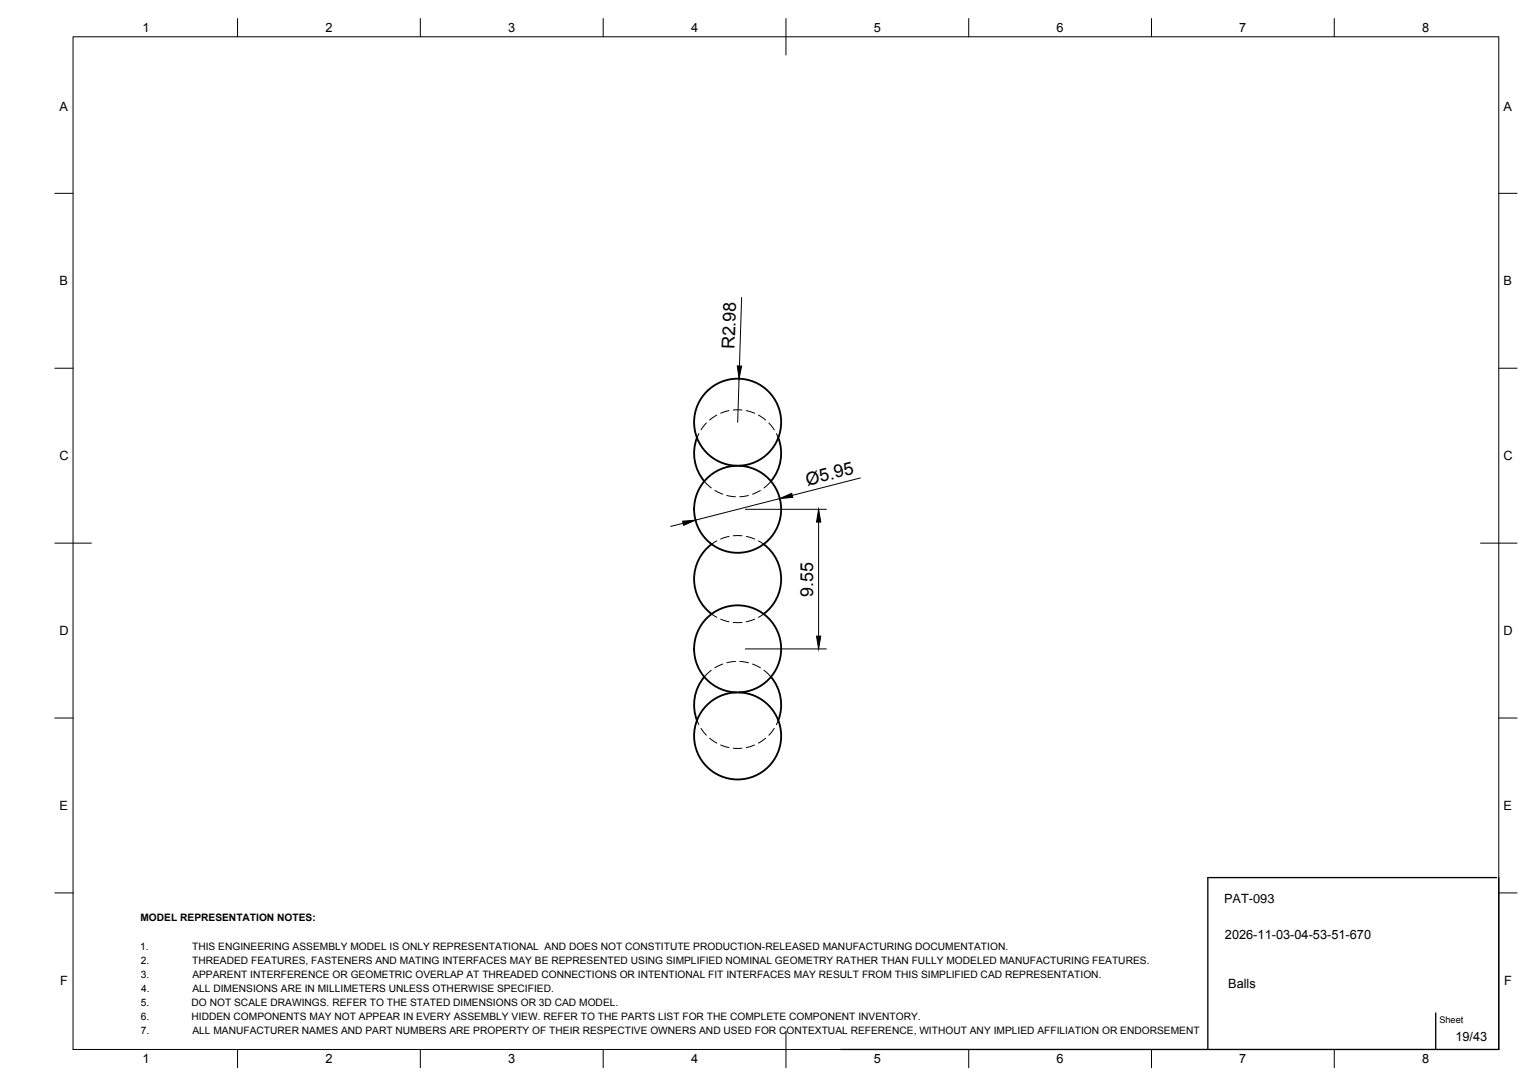
ISO-10303-21;
HEADER;
/* Generated by software containing ST-Developer
 * from STEP Tools, Inc. (www.steptools.com) 
 */

FILE_DESCRIPTION(
/* description */ ('Self-centering screw clamp'),
/* implementation_level */ '2;1');

FILE_NAME(
/* name */ 'Balls.step',
/* time_stamp */ '2026-10-28T03:25:31-07:00',
/* author */ (''),
/* organization */ (''),
/* preprocessor_version */ 'ST-DEVELOPER v20.2',
/* originating_system */ 'Autodesk Translation Framework v15.17.0.0',
/* authorisation */ '');

FILE_SCHEMA (('AUTOMOTIVE_DESIGN { 1 0 10303 214 3 1 1 }'));
ENDSEC;

DATA;
#10=MECHANICAL_DESIGN_GEOMETRIC_PRESENTATION_REPRESENTATION('',(#640,#641,#642,#643,#644,#645,#646),#16799);
#467=SPHERICAL_SURFACE('',#9996,0.29765);
#468=SPHERICAL_SURFACE('',#9998,0.29765);
#469=SPHERICAL_SURFACE('',#10000,0.29765);
#470=SPHERICAL_SURFACE('',#10002,0.29765);
#471=SPHERICAL_SURFACE('',#10004,0.29765);
#472=SPHERICAL_SURFACE('',#10006,0.29765);
#473=SPHERICAL_SURFACE('',#10008,0.29765);
#558=SHAPE_REPRESENTATION_RELATIONSHIP('SRR','None',#17032,#599);
#599=ADVANCED_BREP_SHAPE_REPRESENTATION('',(#688,#689,#690,#691,#692,#693,
#694),#16770);
#640=STYLED_ITEM('',(#17326),#688);
#641=STYLED_ITEM('',(#17326),#689);
#642=STYLED_ITEM('',(#17326),#690);
#643=STYLED_ITEM('',(#17326),#691);
#644=STYLED_ITEM('',(#17326),#692);
#645=STYLED_ITEM('',(#17326),#693);
#646=STYLED_ITEM('',(#17326),#694);
#688=MANIFOLD_SOLID_BREP('Body1',#9091);
#689=MANIFOLD_SOLID_BREP('Body2',#9092);
#690=MANIFOLD_SOLID_BREP('Body3',#9093);
#691=MANIFOLD_SOLID_BREP('Body4',#9094);
#692=MANIFOLD_SOLID_BREP('Body5',#9095);
#693=MANIFOLD_SOLID_BREP('Body6',#9096);
#694=MANIFOLD_SOLID_BREP('Body7',#9097);
#1470=FACE_OUTER_BOUND('',#2102,.T.);
#1471=FACE_OUTER_BOUND('',#2103,.T.);
#1472=FACE_OUTER_BOUND('',#2104,.T.);
#1473=FACE_OUTER_BOUND('',#2105,.T.);
#1474=FACE_OUTER_BOUND('',#2106,.T.);
#1475=FACE_OUTER_BOUND('',#2107,.T.);
#1476=FACE_OUTER_BOUND('',#2108,.T.);
#2102=EDGE_LOOP('',(#7057,#7058));
#2103=EDGE_LOOP('',(#7059,#7060));
#2104=EDGE_LOOP('',(#7061,#7062));
#2105=EDGE_LOOP('',(#7063,#7064));
#2106=EDGE_LOOP('',(#7065,#7066));
#2107=EDGE_LOOP('',(#7067,#7068));
#2108=EDGE_LOOP('',(#7069,#7070));
#3925=CIRCLE('',#9997,0.29765);
#3926=CIRCLE('',#9999,0.29765);
#3927=CIRCLE('',#10001,0.29765);
#3928=CIRCLE('',#10003,0.29765);
#3929=CIRCLE('',#10005,0.29765);
#3930=CIRCLE('',#10007,0.29765);
#3931=CIRCLE('',#10009,0.29765);
#4537=VERTEX_POINT('',#14754);
#4538=VERTEX_POINT('',#14755);
#4539=VERTEX_POINT('',#14758);
#4540=VERTEX_POINT('',#14759);
#4541=VERTEX_POINT('',#14762);
#4542=VERTEX_POINT('',#14763);
#4543=VERTEX_POINT('',#14766);
#4544=VERTEX_POINT('',#14767);
#4545=VERTEX_POINT('',#14770);
#4546=VERTEX_POINT('',#14771);
#4547=VERTEX_POINT('',#14774);
#4548=VERTEX_POINT('',#14775);
#4549=VERTEX_POINT('',#14778);
#4550=VERTEX_POINT('',#14779);
#5453=EDGE_CURVE('',#4537,#4538,#3925,.T.);
#5454=EDGE_CURVE('',#4539,#4540,#3926,.T.);
#5455=EDGE_CURVE('',#4541,#4542,#3927,.T.);
#5456=EDGE_CURVE('',#4543,#4544,#3928,.T.);
#5457=EDGE_CURVE('',#4545,#4546,#3929,.T.);
#5458=EDGE_CURVE('',#4547,#4548,#3930,.T.);
#5459=EDGE_CURVE('',#4549,#4550,#3931,.T.);
#7057=ORIENTED_EDGE('',*,*,#5453,.T.);
#7058=ORIENTED_EDGE('',*,*,#5453,.F.);
#7059=ORIENTED_EDGE('',*,*,#5454,.T.);
#7060=ORIENTED_EDGE('',*,*,#5454,.F.);
#7061=ORIENTED_EDGE('',*,*,#5455,.T.);
#7062=ORIENTED_EDGE('',*,*,#5455,.F.);
#7063=ORIENTED_EDGE('',*,*,#5456,.T.);
#7064=ORIENTED_EDGE('',*,*,#5456,.F.);
#7065=ORIENTED_EDGE('',*,*,#5457,.T.);
#7066=ORIENTED_EDGE('',*,*,#5457,.F.);
#7067=ORIENTED_EDGE('',*,*,#5458,.T.);
#7068=ORIENTED_EDGE('',*,*,#5458,.F.);
#7069=ORIENTED_EDGE('',*,*,#5459,.T.);
#7070=ORIENTED_EDGE('',*,*,#5459,.F.);
#8768=ADVANCED_FACE('',(#1470),#467,.T.);
#8769=ADVANCED_FACE('',(#1471),#468,.T.);
#8770=ADVANCED_FACE('',(#1472),#469,.T.);
#8771=ADVANCED_FACE('',(#1473),#470,.T.);
#8772=ADVANCED_FACE('',(#1474),#471,.T.);
#8773=ADVANCED_FACE('',(#1475),#472,.T.);
#8774=ADVANCED_FACE('',(#1476),#473,.T.);
#9091=CLOSED_SHELL('',(#8768));
#9092=CLOSED_SHELL('',(#8769));
#9093=CLOSED_SHELL('',(#8770));
#9094=CLOSED_SHELL('',(#8771));
#9095=CLOSED_SHELL('',(#8772));
#9096=CLOSED_SHELL('',(#8773));
#9097=CLOSED_SHELL('',(#8774));
#9995=AXIS2_PLACEMENT_3D('',#14752,#11847,#11848);
#9996=AXIS2_PLACEMENT_3D('',#14753,#11849,#11850);
#9997=AXIS2_PLACEMENT_3D('',#14756,#11851,#11852);
#9998=AXIS2_PLACEMENT_3D('',#14757,#11853,#11854);
#9999=AXIS2_PLACEMENT_3D('',#14760,#11855,#11856);
#10000=AXIS2_PLACEMENT_3D('',#14761,#11857,#11858);
#10001=AXIS2_PLACEMENT_3D('',#14764,#11859,#11860);
#10002=AXIS2_PLACEMENT_3D('',#14765,#11861,#11862);
#10003=AXIS2_PLACEMENT_3D('',#14768,#11863,#11864);
#10004=AXIS2_PLACEMENT_3D('',#14769,#11865,#11866);
#10005=AXIS2_PLACEMENT_3D('',#14772,#11867,#11868);
#10006=AXIS2_PLACEMENT_3D('',#14773,#11869,#11870);
#10007=AXIS2_PLACEMENT_3D('',#14776,#11871,#11872);
#10008=AXIS2_PLACEMENT_3D('',#14777,#11873,#11874);
#10009=AXIS2_PLACEMENT_3D('',#14780,#11875,#11876);
#11847=DIRECTION('axis',(0.,0.,1.));
#11848=DIRECTION('refdir',(1.,0.,0.));
#11849=DIRECTION('center_axis',(0.,0.,1.));
#11850=DIRECTION('ref_axis',(1.,0.,0.));
#11851=DIRECTION('center_axis',(1.22464679914735E-16,-1.,0.));
#11852=DIRECTION('ref_axis',(-1.,-1.22464679914735E-16,0.));
#11853=DIRECTION('center_axis',(0.78183148246803,0.,0.623489801858733));
#11854=DIRECTION('ref_axis',(0.623489801858734,0.,-0.78183148246803));
#11855=DIRECTION('center_axis',(7.63554790147315E-17,-1.,-9.57467422477103E-17));
#11856=DIRECTION('ref_axis',(-0.623489801858734,-1.22464679914735E-16,0.78183148246803));
#11857=DIRECTION('center_axis',(0.974927912181824,0.,-0.222520933956314));
#11858=DIRECTION('ref_axis',(-0.222520933956314,0.,-0.974927912181824));
#11859=DIRECTION('center_axis',(-2.7250954951288E-17,-1.,-1.19394234705288E-16));
#11860=DIRECTION('ref_axis',(0.222520933956314,-1.22464679914735E-16,0.974927912181824));
#11861=DIRECTION('center_axis',(0.433883739117558,0.,-0.900968867902419));
#11862=DIRECTION('ref_axis',(-0.900968867902419,0.,-0.433883739117558));
#11863=DIRECTION('center_axis',(-1.10336864020811E-16,-1.,-5.31354332312403E-17));
#11864=DIRECTION('ref_axis',(0.900968867902419,-1.22464679914735E-16,0.433883739117558));
#11865=DIRECTION('center_axis',(-0.433883739117558,0.,-0.900968867902419));
#11866=DIRECTION('ref_axis',(-0.900968867902419,0.,0.433883739117558));
#11867=DIRECTION('center_axis',(-1.10336864020811E-16,-1.,5.31354332312403E-17));
#11868=DIRECTION('ref_axis',(0.900968867902419,-1.22464679914735E-16,-0.433883739117558));
#11869=DIRECTION('center_axis',(-0.974927912181824,0.,-0.222520933956314));
#11870=DIRECTION('ref_axis',(-0.222520933956315,0.,0.974927912181824));
#11871=DIRECTION('center_axis',(-2.7250954951288E-17,-1.,1.19394234705288E-16));
#11872=DIRECTION('ref_axis',(0.222520933956315,-1.22464679914735E-16,-0.974927912181824));
#11873=DIRECTION('center_axis',(-0.78183148246803,0.,0.623489801858734));
#11874=DIRECTION('ref_axis',(0.623489801858733,0.,0.78183148246803));
#11875=DIRECTION('center_axis',(7.63554790147315E-17,-1.,9.57467422477103E-17));
#11876=DIRECTION('ref_axis',(-0.623489801858733,-1.22464679914735E-16,-0.78183148246803));
#14752=CARTESIAN_POINT('',(0.,0.,0.));
#14753=CARTESIAN_POINT('Origin',(1.1,0.,0.));
#14754=CARTESIAN_POINT('',(1.1,-2.23201749654651E-33,0.29765));
#14755=CARTESIAN_POINT('',(1.1,-2.23201749654651E-33,-0.29765));
#14756=CARTESIAN_POINT('Origin',(1.1,0.,0.));
#14757=CARTESIAN_POINT('Origin',(0.685838782044607,0.,-0.860014630714833));
#14758=CARTESIAN_POINT('',(0.918550922801216,-5.31350540756609E-33,-0.674432891191581));
#14759=CARTESIAN_POINT('',(0.453126641287998,8.49470414473068E-34,-1.04559637023808));
#14760=CARTESIAN_POINT('Origin',(0.685838782044607,0.,-0.860014630714833));
#14761=CARTESIAN_POINT('Origin',(-0.244773027351946,0.,-1.07242070340001));
#14762=CARTESIAN_POINT('',(0.0454142657089739,-2.23201749654651E-33,-1.1386540593921));
#14763=CARTESIAN_POINT('',(-0.534960320412865,-2.23201749654651E-33,-1.00618734740791));
#14764=CARTESIAN_POINT('Origin',(-0.244773027351946,0.,-1.07242070340001));
#14765=CARTESIAN_POINT('Origin',(-0.991065754692661,0.,-0.477272113029314));
#14766=CARTESIAN_POINT('',(-0.86192025974432,8.49470414473067E-34,-0.745445496560469));
#14767=CARTESIAN_POINT('',(-1.120211249641,-5.31350540756609E-33,-0.209098729498159));
#14768=CARTESIAN_POINT('Origin',(-0.991065754692661,0.,-0.477272113029314));
#14769=CARTESIAN_POINT('Origin',(-0.991065754692661,0.,0.477272113029314));
#14770=CARTESIAN_POINT('',(-1.120211249641,-2.23201749654651E-33,0.209098729498159));
#14771=CARTESIAN_POINT('',(-0.86192025974432,-2.23201749654651E-33,0.745445496560469));
#14772=CARTESIAN_POINT('Origin',(-0.991065754692661,0.,0.477272113029314));
#14773=CARTESIAN_POINT('Origin',(-0.244773027351946,0.,1.07242070340001));
#14774=CARTESIAN_POINT('',(-0.534960320412866,-2.23201749654651E-33,1.00618734740791));
#14775=CARTESIAN_POINT('',(0.0454142657089737,-2.23201749654651E-33,1.1386540593921));
#14776=CARTESIAN_POINT('Origin',(-0.244773027351946,0.,1.07242070340001));
#14777=CARTESIAN_POINT('Origin',(0.685838782044607,0.,0.860014630714833));
#14778=CARTESIAN_POINT('',(0.453126641287998,-2.23201749654651E-33,1.04559637023808));
#14779=CARTESIAN_POINT('',(0.918550922801216,-2.23201749654651E-33,0.674432891191581));
#14780=CARTESIAN_POINT('Origin',(0.685838782044607,0.,0.860014630714833));
#16721=UNCERTAINTY_MEASURE_WITH_UNIT(LENGTH_MEASURE(0.001),#16800,
'DISTANCE_ACCURACY_VALUE',
'Maximum model space distance between geometric entities at asserted c
onnectivities');
#16750=UNCERTAINTY_MEASURE_WITH_UNIT(LENGTH_MEASURE(0.001),#16800,
'DISTANCE_ACCURACY_VALUE',
'Maximum model space distance between geometric entities at asserted c
onnectivities');
#16770=(
GEOMETRIC_REPRESENTATION_CONTEXT(3)
GLOBAL_UNCERTAINTY_ASSIGNED_CONTEXT((#16721))
GLOBAL_UNIT_ASSIGNED_CONTEXT((#16800,#16802,#16803))
REPRESENTATION_CONTEXT('','3D')
);
#16799=(
GEOMETRIC_REPRESENTATION_CONTEXT(3)
GLOBAL_UNCERTAINTY_ASSIGNED_CONTEXT((#16750))
GLOBAL_UNIT_ASSIGNED_CONTEXT((#16800,#16802,#16803))
REPRESENTATION_CONTEXT('','3D')
);
#16800=(
LENGTH_UNIT()
NAMED_UNIT(*)
SI_UNIT(.CENTI.,.METRE.)
);
#16802=(
NAMED_UNIT(*)
PLANE_ANGLE_UNIT()
SI_UNIT($,.RADIAN.)
);
#16803=(
NAMED_UNIT(*)
SI_UNIT($,.STERADIAN.)
SOLID_ANGLE_UNIT()
);
#16823=SHAPE_DEFINITION_REPRESENTATION(#16871,#17032);
#16871=PRODUCT_DEFINITION_SHAPE('',$,#17081);
#17032=SHAPE_REPRESENTATION('',(#9995),#16770);
#17061=PRODUCT_DEFINITION_CONTEXT('part definition',#17207,'design');
#17081=PRODUCT_DEFINITION('Balls','Balls',#17129,#17061);
#17129=PRODUCT_DEFINITION_FORMATION('',$,#17228);
#17207=APPLICATION_CONTEXT(
'Core Data for Automotive Mechanical Design Process');
#17208=PRODUCT_CONTEXT('part definition',#17207,'mechanical');
#17228=PRODUCT('Balls','Balls','Balls',(#17208));
#17320=COLOUR_RGB('Grey',0.48,0.52,0.57);
#17321=FILL_AREA_STYLE_COLOUR('',#17320);
#17322=FILL_AREA_STYLE('',(#17321));
#17323=SURFACE_STYLE_FILL_AREA(#17322);
#17324=SURFACE_SIDE_STYLE('',(#17323));
#17325=SURFACE_STYLE_USAGE(.BOTH.,#17324);
#17326=PRESENTATION_STYLE_ASSIGNMENT((#17325));
ENDSEC;
END-ISO-10303-21;
